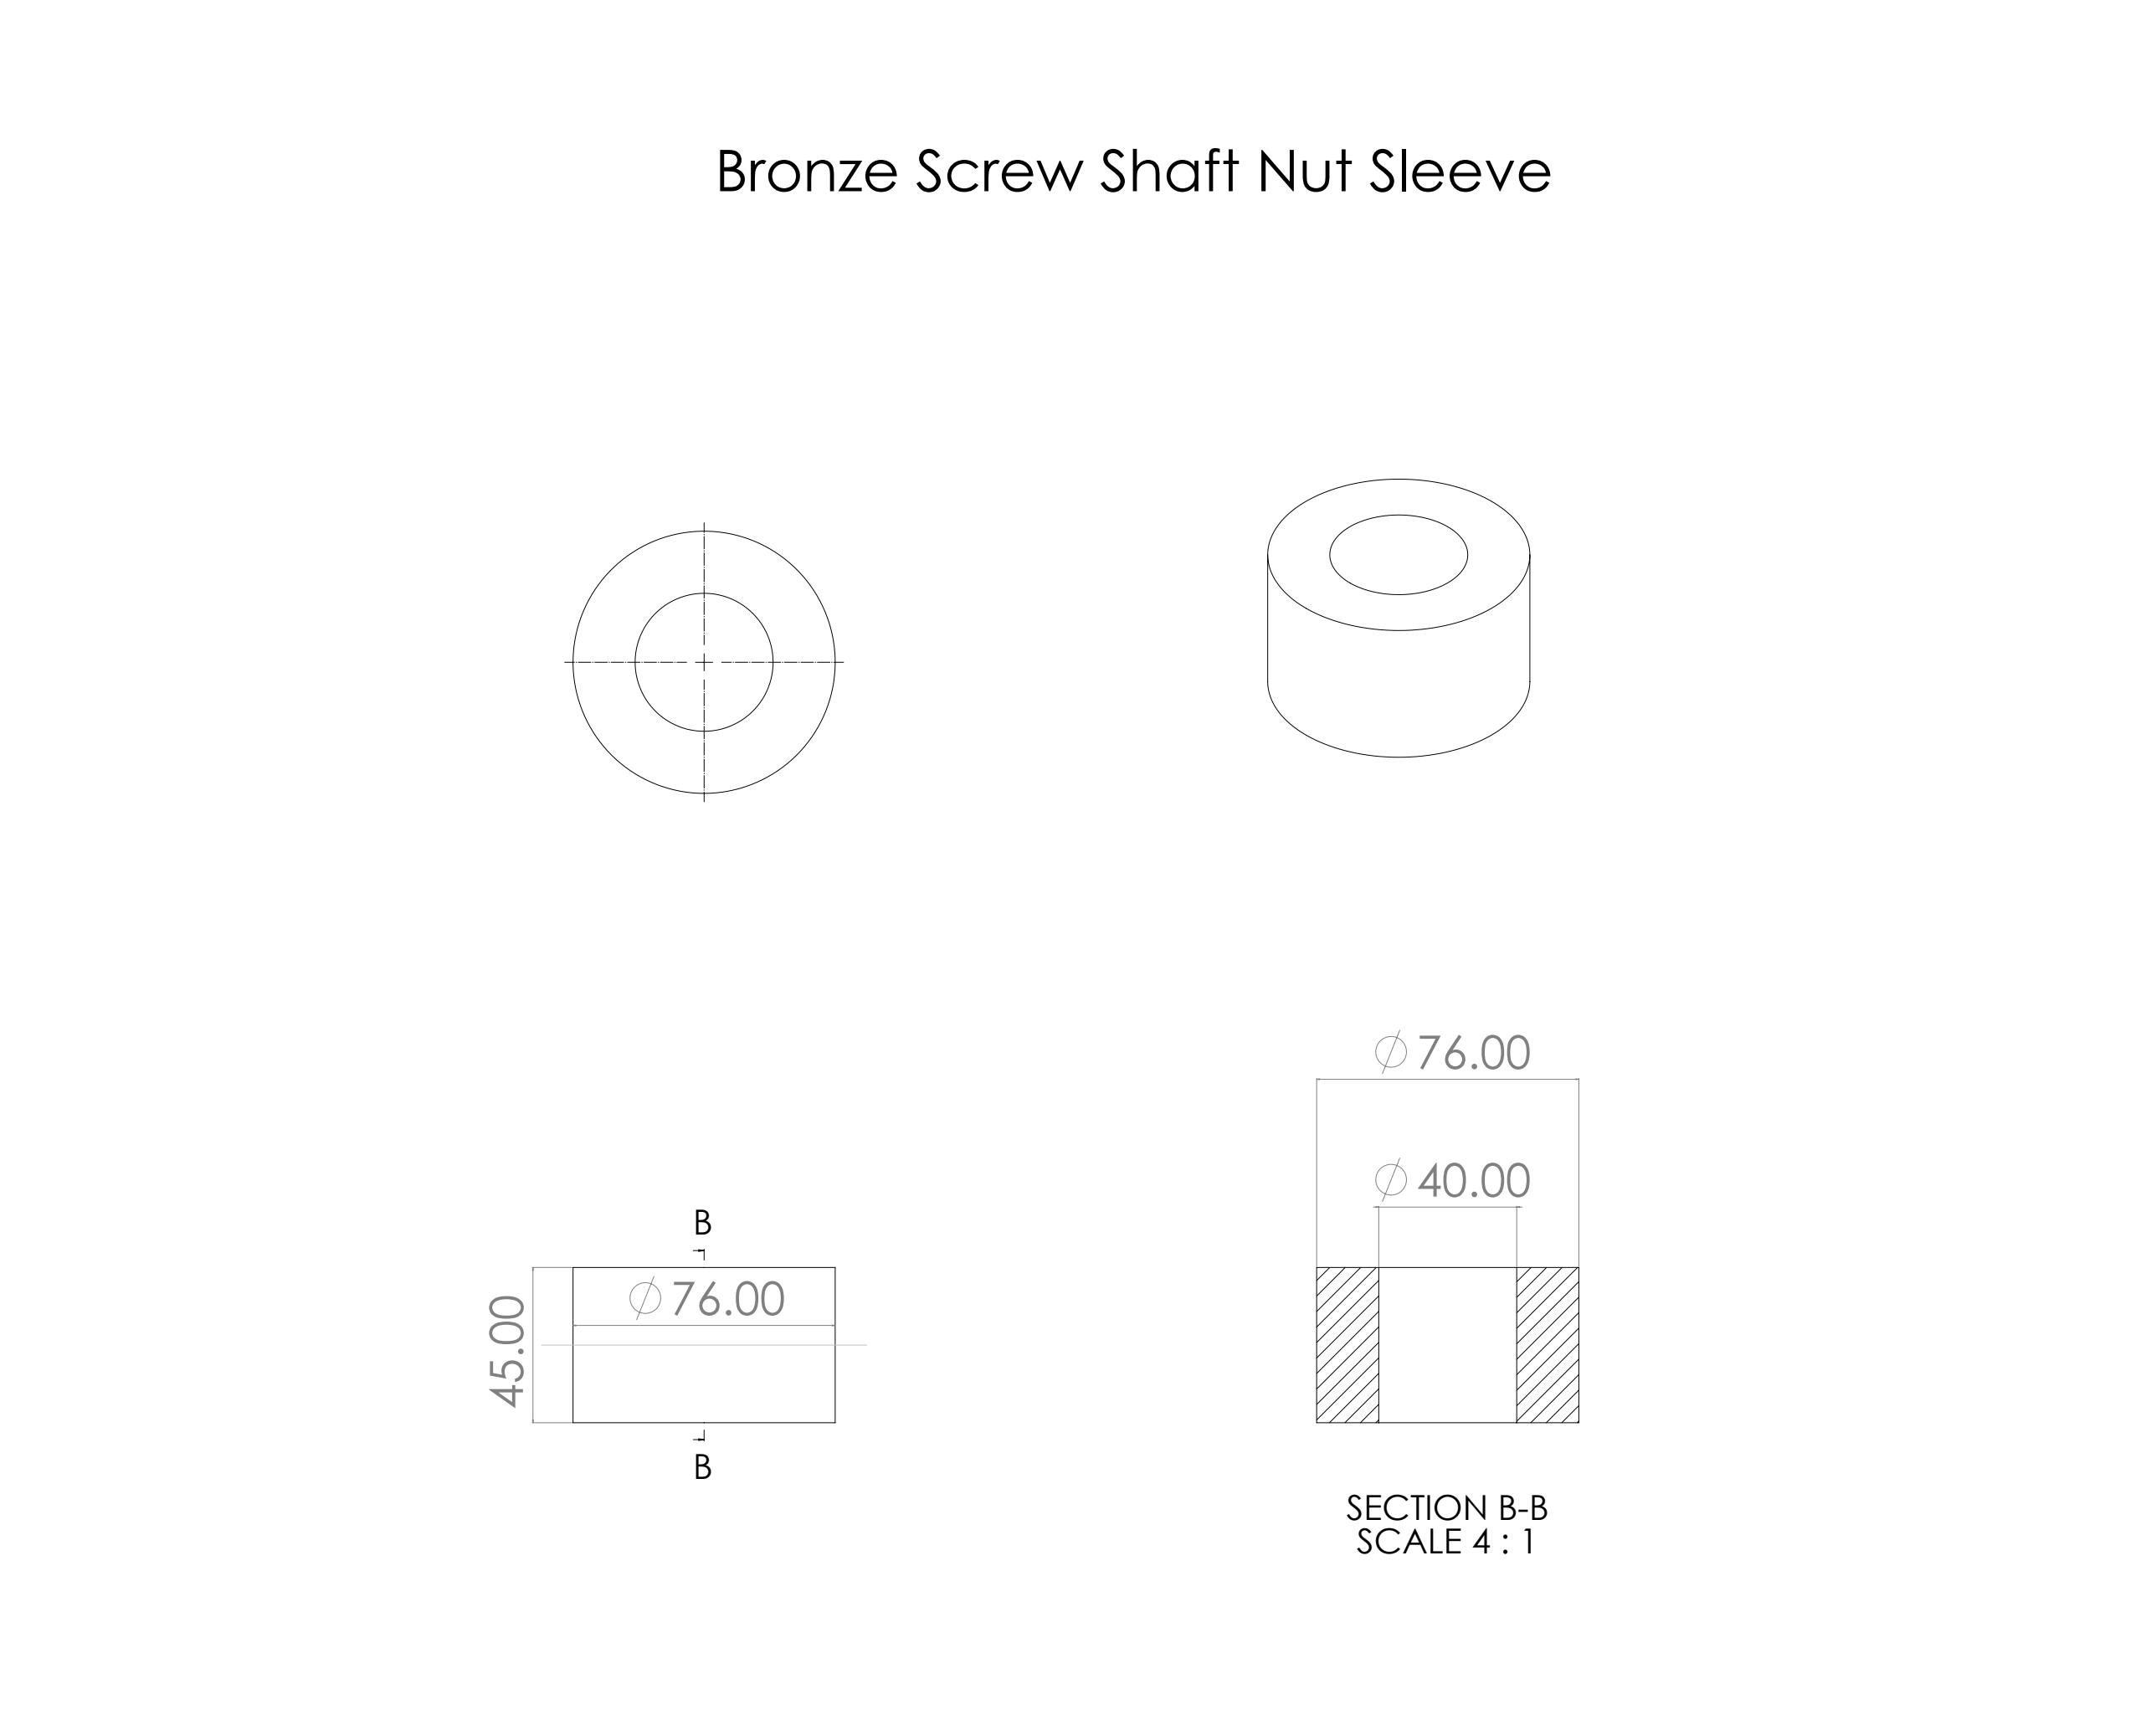
ISO-10303-21;
HEADER;
FILE_DESCRIPTION (('STEP AP214'),
    '1' );
FILE_NAME ('Bronze Screw Shaft Nut Sleeve.step',
    '2026-10-24T00:28:05',
    ( '' ),
    ( '' ),
    'SwSTEP 2.0',
    'SolidWorks 2025',
    '' );
FILE_SCHEMA (( 'AUTOMOTIVE_DESIGN' ));
ENDSEC;

DATA;
#278=DIRECTION ( 'NONE',  ( 0.000000000000000000, 1.000000000000000000, 0.000000000000000000 ) ) ;
#319=DIRECTION ( 'NONE',  ( -0.000000000000000000, -1.000000000000000000, -0.000000000000000000 ) ) ;
#424=VECTOR ( 'NONE', #12547, 1000.000000000000000 ) ;
#498=DIRECTION ( 'NONE',  ( 0.000000000000000000, 1.000000000000000000, 0.000000000000000000 ) ) ;
#618=PLANE ( 'NONE',  #17372 ) ;
#621=( NAMED_UNIT ( * ) SI_UNIT ( $, .STERADIAN. ) SOLID_ANGLE_UNIT ( ) );
#636=ORIENTED_EDGE ( 'NONE', *, *, #9399, .F. ) ;
#655=DIRECTION ( 'NONE',  ( 0.000000000000000000, -0.000000000000000000, 1.000000000000000000 ) ) ;
#669=CARTESIAN_POINT ( 'NONE',  ( -28.68588794268872633, 333.8848358243226357, 0.000000000000000000 ) ) ;
#696=DIRECTION ( 'NONE',  ( 1.000000000000000000, 0.000000000000000000, 0.000000000000000000 ) ) ;
#743=EDGE_LOOP ( 'NONE', ( #12218, #10443, #10130, #5735 ) ) ;
#808=CARTESIAN_POINT ( 'NONE',  ( 0.000000000000000000, 0.000000000000000000, 0.000000000000000000 ) ) ;
#914=( NAMED_UNIT ( * ) PLANE_ANGLE_UNIT ( ) SI_UNIT ( $, .RADIAN. ) );
#1431=DIRECTION ( 'NONE',  ( 0.000000000000000000, 1.000000000000000000, 0.000000000000000000 ) ) ;
#1751=CIRCLE ( 'NONE', #2104, 38.00000000000000000 ) ;
#1895=SHAPE_DEFINITION_REPRESENTATION ( #6296, #10694 ) ;
#2036=CARTESIAN_POINT ( 'NONE',  ( -28.68588794268872633, 333.8848358243226357, -20.00000000000000000 ) ) ;
#2104=AXIS2_PLACEMENT_3D ( 'NONE', #6741, #278, #7476 ) ;
#2288=PRODUCT_DEFINITION_CONTEXT ( 'detailed design', #7359, 'design' ) ;
#2341=( NAMED_UNIT ( * ) PLANE_ANGLE_UNIT ( ) SI_UNIT ( $, .RADIAN. ) );
#2419=DIRECTION ( 'NONE',  ( 0.000000000000000000, 0.000000000000000000, 1.000000000000000000 ) ) ;
#2450=CLOSED_SHELL ( 'NONE', ( #19758, #11324, #20934, #6664, #18208, #6389 ) ) ;
#2482=DIRECTION ( 'NONE',  ( 0.000000000000000000, 1.000000000000000000, 0.000000000000000000 ) ) ;
#2629=SHAPE_REPRESENTATION_RELATIONSHIP ( 'NONE' , 'NONE' ,  #10694, #21324 ) ;
#2700=CARTESIAN_POINT ( 'NONE',  ( -28.68588794268872277, 378.8848358243226357, 38.00000000000000000 ) ) ;
#2980=DIRECTION ( 'NONE',  ( 0.000000000000000000, 1.000000000000000000, 0.000000000000000000 ) ) ;
#3257=CARTESIAN_POINT ( 'NONE',  ( -28.68588794268872633, 378.8848358243226357, 0.000000000000000000 ) ) ;
#3302=CARTESIAN_POINT ( 'NONE',  ( -28.68588794268872633, 378.8848358243226357, 0.000000000000000000 ) ) ;
#3442=CARTESIAN_POINT ( 'NONE',  ( -28.68588794268872633, 378.8848358243226357, 0.000000000000000000 ) ) ;
#3832=EDGE_CURVE ( 'NONE', #12194, #17559, #1751, .T. ) ;
#4000=UNCERTAINTY_MEASURE_WITH_UNIT (LENGTH_MEASURE( 1.000000000000000082E-05 ), #7374, 'distance_accuracy_value', 'NONE');
#4176=DIRECTION ( 'NONE',  ( -0.000000000000000000, -1.000000000000000000, -0.000000000000000000 ) ) ;
#4422=EDGE_LOOP ( 'NONE', ( #13095, #13480 ) ) ;
#4471=AXIS2_PLACEMENT_3D ( 'NONE', #9738, #1431, #17959 ) ;
#4503=ORIENTED_EDGE ( 'NONE', *, *, #3832, .T. ) ;
#4508=MANIFOLD_SOLID_BREP ( 'Boss-Extrude6', #2450 ) ;
#4632=ORIENTED_EDGE ( 'NONE', *, *, #14597, .F. ) ;
#4707=EDGE_LOOP ( 'NONE', ( #6643, #4951, #636, #18935 ) ) ;
#4951=ORIENTED_EDGE ( 'NONE', *, *, #6962, .T. ) ;
#5516=DIRECTION ( 'NONE',  ( 0.000000000000000000, 1.000000000000000000, 0.000000000000000000 ) ) ;
#5571=DIRECTION ( 'NONE',  ( 0.000000000000000000, 1.000000000000000000, 0.000000000000000000 ) ) ;
#5735=ORIENTED_EDGE ( 'NONE', *, *, #20130, .F. ) ;
#5795=CARTESIAN_POINT ( 'NONE',  ( -28.68588794268872633, 378.8848358243226357, -38.00000000000000000 ) ) ;
#6040=LINE ( 'NONE', #12323, #424 ) ;
#6296=PRODUCT_DEFINITION_SHAPE ( 'NONE', 'NONE',  #18472 ) ;
#6377=CARTESIAN_POINT ( 'NONE',  ( -28.68588794268872633, 378.8848358243226357, -20.00000000000000000 ) ) ;
#6389=ADVANCED_FACE ( 'NONE', ( #19680 ), #6906, .F. ) ;
#6416=CIRCLE ( 'NONE', #7467, 20.00000000000000000 ) ;
#6643=ORIENTED_EDGE ( 'NONE', *, *, #12867, .T. ) ;
#6664=ADVANCED_FACE ( 'NONE', ( #18692, #14063 ), #15470, .F. ) ;
#6741=CARTESIAN_POINT ( 'NONE',  ( -28.68588794268872633, 333.8848358243226357, 0.000000000000000000 ) ) ;
#6781=CYLINDRICAL_SURFACE ( 'NONE', #14591, 38.00000000000000000 ) ;
#6826=VERTEX_POINT ( 'NONE', #2700 ) ;
#6906=CYLINDRICAL_SURFACE ( 'NONE', #9433, 20.00000000000000000 ) ;
#6962=EDGE_CURVE ( 'NONE', #9177, #20205, #9705, .T. ) ;
#6994=DIRECTION ( 'NONE',  ( 0.000000000000000000, 0.000000000000000000, -1.000000000000000000 ) ) ;
#7013=ORIENTED_EDGE ( 'NONE', *, *, #12867, .F. ) ;
#7203=VECTOR ( 'NONE', #12360, 1000.000000000000000 ) ;
#7235=DIRECTION ( 'NONE',  ( 0.000000000000000000, 0.000000000000000000, 1.000000000000000000 ) ) ;
#7345=DIRECTION ( 'NONE',  ( 0.000000000000000000, 0.000000000000000000, 1.000000000000000000 ) ) ;
#7355=ORIENTED_EDGE ( 'NONE', *, *, #17106, .T. ) ;
#7359=APPLICATION_CONTEXT ( 'automotive_design' ) ;
#7374=( LENGTH_UNIT ( ) NAMED_UNIT ( * ) SI_UNIT ( .MILLI., .METRE. ) );
#7407=FACE_OUTER_BOUND ( 'NONE', #20977, .T. ) ;
#7436=ORIENTED_EDGE ( 'NONE', *, *, #7586, .F. ) ;
#7467=AXIS2_PLACEMENT_3D ( 'NONE', #3302, #9875, #13031 ) ;
#7476=DIRECTION ( 'NONE',  ( 0.000000000000000000, 0.000000000000000000, 1.000000000000000000 ) ) ;
#7586=EDGE_CURVE ( 'NONE', #19261, #17559, #20619, .T. ) ;
#7928=DIRECTION ( 'NONE',  ( 0.000000000000000000, 0.000000000000000000, 1.000000000000000000 ) ) ;
#8034=FACE_OUTER_BOUND ( 'NONE', #4707, .T. ) ;
#8092=UNCERTAINTY_MEASURE_WITH_UNIT (LENGTH_MEASURE( 1.000000000000000082E-05 ), #20718, 'distance_accuracy_value', 'NONE');
#8323=AXIS2_PLACEMENT_3D ( 'NONE', #3257, #16353, #9834 ) ;
#8361=STYLED_ITEM('',(#21442),#4508);
#8375=ORIENTED_EDGE ( 'NONE', *, *, #15894, .F. ) ;
#8419=CARTESIAN_POINT ( 'NONE',  ( -28.68588794268872633, 333.8848358243226357, -38.00000000000000000 ) ) ;
#8427=DIRECTION ( 'NONE',  ( -0.000000000000000000, -1.000000000000000000, -0.000000000000000000 ) ) ;
#8515=AXIS2_PLACEMENT_3D ( 'NONE', #15656, #10759, #15759 ) ;
#8591=EDGE_LOOP ( 'NONE', ( #8375, #20765, #4503, #7436 ) ) ;
#9082=DIRECTION ( 'NONE',  ( 0.000000000000000000, 1.000000000000000000, 0.000000000000000000 ) ) ;
#9177=VERTEX_POINT ( 'NONE', #18522 ) ;
#9217=EDGE_CURVE ( 'NONE', #10520, #13969, #18838, .T. ) ;
#9350=CARTESIAN_POINT ( 'NONE',  ( -28.68588794268872633, 378.8848358243226357, 0.000000000000000000 ) ) ;
#9399=EDGE_CURVE ( 'NONE', #13969, #20205, #21040, .T. ) ;
#9433=AXIS2_PLACEMENT_3D ( 'NONE', #13208, #8427, #16671 ) ;
#9556=DIRECTION ( 'NONE',  ( 0.000000000000000000, 0.000000000000000000, -1.000000000000000000 ) ) ;
#9705=LINE ( 'NONE', #11434, #11865 ) ;
#9738=CARTESIAN_POINT ( 'NONE',  ( -28.68588794268872633, 333.8848358243226357, 0.000000000000000000 ) ) ;
#9834=DIRECTION ( 'NONE',  ( 0.000000000000000000, 0.000000000000000000, 1.000000000000000000 ) ) ;
#9875=DIRECTION ( 'NONE',  ( 0.000000000000000000, 1.000000000000000000, 0.000000000000000000 ) ) ;
#10026=FACE_OUTER_BOUND ( 'NONE', #8591, .T. ) ;
#10130=ORIENTED_EDGE ( 'NONE', *, *, #9217, .T. ) ;
#10133=AXIS2_PLACEMENT_3D ( 'NONE', #14665, #19513, #9556 ) ;
#10180=ORIENTED_EDGE ( 'NONE', *, *, #17106, .F. ) ;
#10443=ORIENTED_EDGE ( 'NONE', *, *, #10549, .T. ) ;
#10516=DIRECTION ( 'NONE',  ( 0.000000000000000000, 0.000000000000000000, 1.000000000000000000 ) ) ;
#10520=VERTEX_POINT ( 'NONE', #6377 ) ;
#10549=EDGE_CURVE ( 'NONE', #9177, #10520, #12834, .T. ) ;
#10625=CARTESIAN_POINT ( 'NONE',  ( -28.68588794268872633, 378.8848358243226357, 0.000000000000000000 ) ) ;
#10694=SHAPE_REPRESENTATION ( 'Bronze Screw Shaft Nut Sleeve', ( #12794 ), #14893 ) ;
#10759=DIRECTION ( 'NONE',  ( -0.000000000000000000, -1.000000000000000000, -0.000000000000000000 ) ) ;
#10800=ORIENTED_EDGE ( 'NONE', *, *, #10876, .F. ) ;
#10836=( NAMED_UNIT ( * ) SI_UNIT ( $, .STERADIAN. ) SOLID_ANGLE_UNIT ( ) );
#10876=EDGE_CURVE ( 'NONE', #6826, #12194, #6040, .T. ) ;
#11068=PRODUCT_DEFINITION_FORMATION_WITH_SPECIFIED_SOURCE ( 'ANY', '', #19604, .NOT_KNOWN. ) ;
#11324=ADVANCED_FACE ( 'NONE', ( #10026 ), #6781, .T. ) ;
#11434=CARTESIAN_POINT ( 'NONE',  ( -28.68588794268872277, 378.8848358243226357, 20.00000000000000000 ) ) ;
#11464=( GEOMETRIC_REPRESENTATION_CONTEXT ( 3 ) GLOBAL_UNCERTAINTY_ASSIGNED_CONTEXT ( ( #8092 ) ) GLOBAL_UNIT_ASSIGNED_CONTEXT ( ( #20718, #2341, #621 ) ) REPRESENTATION_CONTEXT ( 'NONE', 'WORKASPACE' ) );
#11818=CARTESIAN_POINT ( 'NONE',  ( -28.68588794268872277, 333.8848358243226357, 38.00000000000000000 ) ) ;
#11865=VECTOR ( 'NONE', #19876, 1000.000000000000000 ) ;
#11926=PRODUCT_CONTEXT ( 'NONE', #16890, 'mechanical' ) ;
#12194=VERTEX_POINT ( 'NONE', #11818 ) ;
#12218=ORIENTED_EDGE ( 'NONE', *, *, #6962, .F. ) ;
#12255=CARTESIAN_POINT ( 'NONE',  ( -28.68588794268872633, 378.8848358243226357, -20.00000000000000000 ) ) ;
#12323=CARTESIAN_POINT ( 'NONE',  ( -28.68588794268872277, 378.8848358243226357, 38.00000000000000000 ) ) ;
#12360=DIRECTION ( 'NONE',  ( -0.000000000000000000, -1.000000000000000000, -0.000000000000000000 ) ) ;
#12547=DIRECTION ( 'NONE',  ( -0.000000000000000000, -1.000000000000000000, -0.000000000000000000 ) ) ;
#12752=ORIENTED_EDGE ( 'NONE', *, *, #9399, .T. ) ;
#12794=AXIS2_PLACEMENT_3D ( 'NONE', #808, #2419, #696 ) ;
#12834=CIRCLE ( 'NONE', #8323, 20.00000000000000000 ) ;
#12867=EDGE_CURVE ( 'NONE', #10520, #9177, #6416, .T. ) ;
#13031=DIRECTION ( 'NONE',  ( 0.000000000000000000, 0.000000000000000000, 1.000000000000000000 ) ) ;
#13095=ORIENTED_EDGE ( 'NONE', *, *, #14597, .T. ) ;
#13136=CYLINDRICAL_SURFACE ( 'NONE', #10133, 20.00000000000000000 ) ;
#13165=CARTESIAN_POINT ( 'NONE',  ( -28.68588794268872633, 378.8848358243226357, -38.00000000000000000 ) ) ;
#13208=CARTESIAN_POINT ( 'NONE',  ( -28.68588794268872633, 378.8848358243226357, 0.000000000000000000 ) ) ;
#13480=ORIENTED_EDGE ( 'NONE', *, *, #15894, .T. ) ;
#13969=VERTEX_POINT ( 'NONE', #2036 ) ;
#14013=ORIENTED_EDGE ( 'NONE', *, *, #7586, .T. ) ;
#14033=CYLINDRICAL_SURFACE ( 'NONE', #8515, 38.00000000000000000 ) ;
#14063=FACE_BOUND ( 'NONE', #19160, .T. ) ;
#14074=CIRCLE ( 'NONE', #19929, 38.00000000000000000 ) ;
#14242=FACE_OUTER_BOUND ( 'NONE', #4422, .T. ) ;
#14297=CARTESIAN_POINT ( 'NONE',  ( -28.68588794268872277, 333.8848358243226357, 20.00000000000000000 ) ) ;
#14438=AXIS2_PLACEMENT_3D ( 'NONE', #20779, #9082, #7345 ) ;
#14571=EDGE_LOOP ( 'NONE', ( #7013, #16830 ) ) ;
#14591=AXIS2_PLACEMENT_3D ( 'NONE', #3442, #319, #6994 ) ;
#14597=EDGE_CURVE ( 'NONE', #19261, #6826, #14074, .T. ) ;
#14665=CARTESIAN_POINT ( 'NONE',  ( -28.68588794268872633, 378.8848358243226357, 0.000000000000000000 ) ) ;
#14757=EDGE_LOOP ( 'NONE', ( #10180, #16858 ) ) ;
#14893=( GEOMETRIC_REPRESENTATION_CONTEXT ( 3 ) GLOBAL_UNCERTAINTY_ASSIGNED_CONTEXT ( ( #4000 ) ) GLOBAL_UNIT_ASSIGNED_CONTEXT ( ( #7374, #914, #10836 ) ) REPRESENTATION_CONTEXT ( 'NONE', 'WORKASPACE' ) );
#15470=PLANE ( 'NONE',  #18063 ) ;
#15656=CARTESIAN_POINT ( 'NONE',  ( -28.68588794268872633, 378.8848358243226357, 0.000000000000000000 ) ) ;
#15759=DIRECTION ( 'NONE',  ( 0.000000000000000000, 0.000000000000000000, -1.000000000000000000 ) ) ;
#15894=EDGE_CURVE ( 'NONE', #6826, #19261, #18891, .T. ) ;
#16353=DIRECTION ( 'NONE',  ( 0.000000000000000000, 1.000000000000000000, 0.000000000000000000 ) ) ;
#16372=CIRCLE ( 'NONE', #19130, 20.00000000000000000 ) ;
#16671=DIRECTION ( 'NONE',  ( 0.000000000000000000, 0.000000000000000000, -1.000000000000000000 ) ) ;
#16830=ORIENTED_EDGE ( 'NONE', *, *, #10549, .F. ) ;
#16858=ORIENTED_EDGE ( 'NONE', *, *, #3832, .F. ) ;
#16890=APPLICATION_CONTEXT ( 'automotive_design' ) ;
#17106=EDGE_CURVE ( 'NONE', #17559, #12194, #21319, .T. ) ;
#17298=CARTESIAN_POINT ( 'NONE',  ( -28.68588794268872633, 333.8848358243226357, 0.000000000000000000 ) ) ;
#17372=AXIS2_PLACEMENT_3D ( 'NONE', #20507, #5571, #19093 ) ;
#17559=VERTEX_POINT ( 'NONE', #8419 ) ;
#17959=DIRECTION ( 'NONE',  ( 0.000000000000000000, 0.000000000000000000, 1.000000000000000000 ) ) ;
#18030=MECHANICAL_DESIGN_GEOMETRIC_PRESENTATION_REPRESENTATION('',(#8361),#11464);
#18063=AXIS2_PLACEMENT_3D ( 'NONE', #17298, #2482, #655 ) ;
#18208=ADVANCED_FACE ( 'NONE', ( #7407 ), #14033, .T. ) ;
#18472=PRODUCT_DEFINITION ( 'UNKNOWN', '', #11068, #2288 ) ;
#18522=CARTESIAN_POINT ( 'NONE',  ( -28.68588794268872277, 378.8848358243226357, 20.00000000000000000 ) ) ;
#18535=AXIS2_PLACEMENT_3D ( 'NONE', #9350, #2980, #7928 ) ;
#18692=FACE_OUTER_BOUND ( 'NONE', #14757, .T. ) ;
#18763=FACE_BOUND ( 'NONE', #14571, .T. ) ;
#18838=LINE ( 'NONE', #12255, #7203 ) ;
#18891=CIRCLE ( 'NONE', #18535, 38.00000000000000000 ) ;
#18932=ORIENTED_EDGE ( 'NONE', *, *, #20130, .T. ) ;
#18935=ORIENTED_EDGE ( 'NONE', *, *, #9217, .F. ) ;
#19093=DIRECTION ( 'NONE',  ( 0.000000000000000000, -0.000000000000000000, 1.000000000000000000 ) ) ;
#19130=AXIS2_PLACEMENT_3D ( 'NONE', #669, #5516, #7235 ) ;
#19160=EDGE_LOOP ( 'NONE', ( #12752, #18932 ) ) ;
#19261=VERTEX_POINT ( 'NONE', #13165 ) ;
#19513=DIRECTION ( 'NONE',  ( -0.000000000000000000, -1.000000000000000000, -0.000000000000000000 ) ) ;
#19604=PRODUCT ( 'Bronze Screw Shaft Nut Sleeve', 'Bronze Screw Shaft Nut Sleeve', '', ( #11926 ) ) ;
#19680=FACE_OUTER_BOUND ( 'NONE', #743, .T. ) ;
#19758=ADVANCED_FACE ( 'NONE', ( #8034 ), #13136, .F. ) ;
#19876=DIRECTION ( 'NONE',  ( -0.000000000000000000, -1.000000000000000000, -0.000000000000000000 ) ) ;
#19929=AXIS2_PLACEMENT_3D ( 'NONE', #10625, #498, #10516 ) ;
#19992=VECTOR ( 'NONE', #4176, 1000.000000000000000 ) ;
#20130=EDGE_CURVE ( 'NONE', #20205, #13969, #16372, .T. ) ;
#20205=VERTEX_POINT ( 'NONE', #14297 ) ;
#20507=CARTESIAN_POINT ( 'NONE',  ( -28.68588794268872633, 378.8848358243226357, 0.000000000000000000 ) ) ;
#20619=LINE ( 'NONE', #5795, #19992 ) ;
#20718=( LENGTH_UNIT ( ) NAMED_UNIT ( * ) SI_UNIT ( .MILLI., .METRE. ) );
#20765=ORIENTED_EDGE ( 'NONE', *, *, #10876, .T. ) ;
#20779=CARTESIAN_POINT ( 'NONE',  ( -28.68588794268872633, 333.8848358243226357, 0.000000000000000000 ) ) ;
#20934=ADVANCED_FACE ( 'NONE', ( #14242, #18763 ), #618, .T. ) ;
#20977=EDGE_LOOP ( 'NONE', ( #10800, #4632, #14013, #7355 ) ) ;
#21040=CIRCLE ( 'NONE', #4471, 20.00000000000000000 ) ;
#21319=CIRCLE ( 'NONE', #14438, 38.00000000000000000 ) ;
#21324=ADVANCED_BREP_SHAPE_REPRESENTATION ( '', ( #4508, #12794 ), #14893 ) ;
#21436=COLOUR_RGB('Black',0.12,0.14,0.17);
#21437=FILL_AREA_STYLE_COLOUR('',#21436);
#21438=FILL_AREA_STYLE('',(#21437));
#21439=SURFACE_STYLE_FILL_AREA(#21438);
#21440=SURFACE_SIDE_STYLE('',(#21439));
#21441=SURFACE_STYLE_USAGE(.BOTH.,#21440);
#21442=PRESENTATION_STYLE_ASSIGNMENT((#21441));
ENDSEC;
END-ISO-10303-21;
